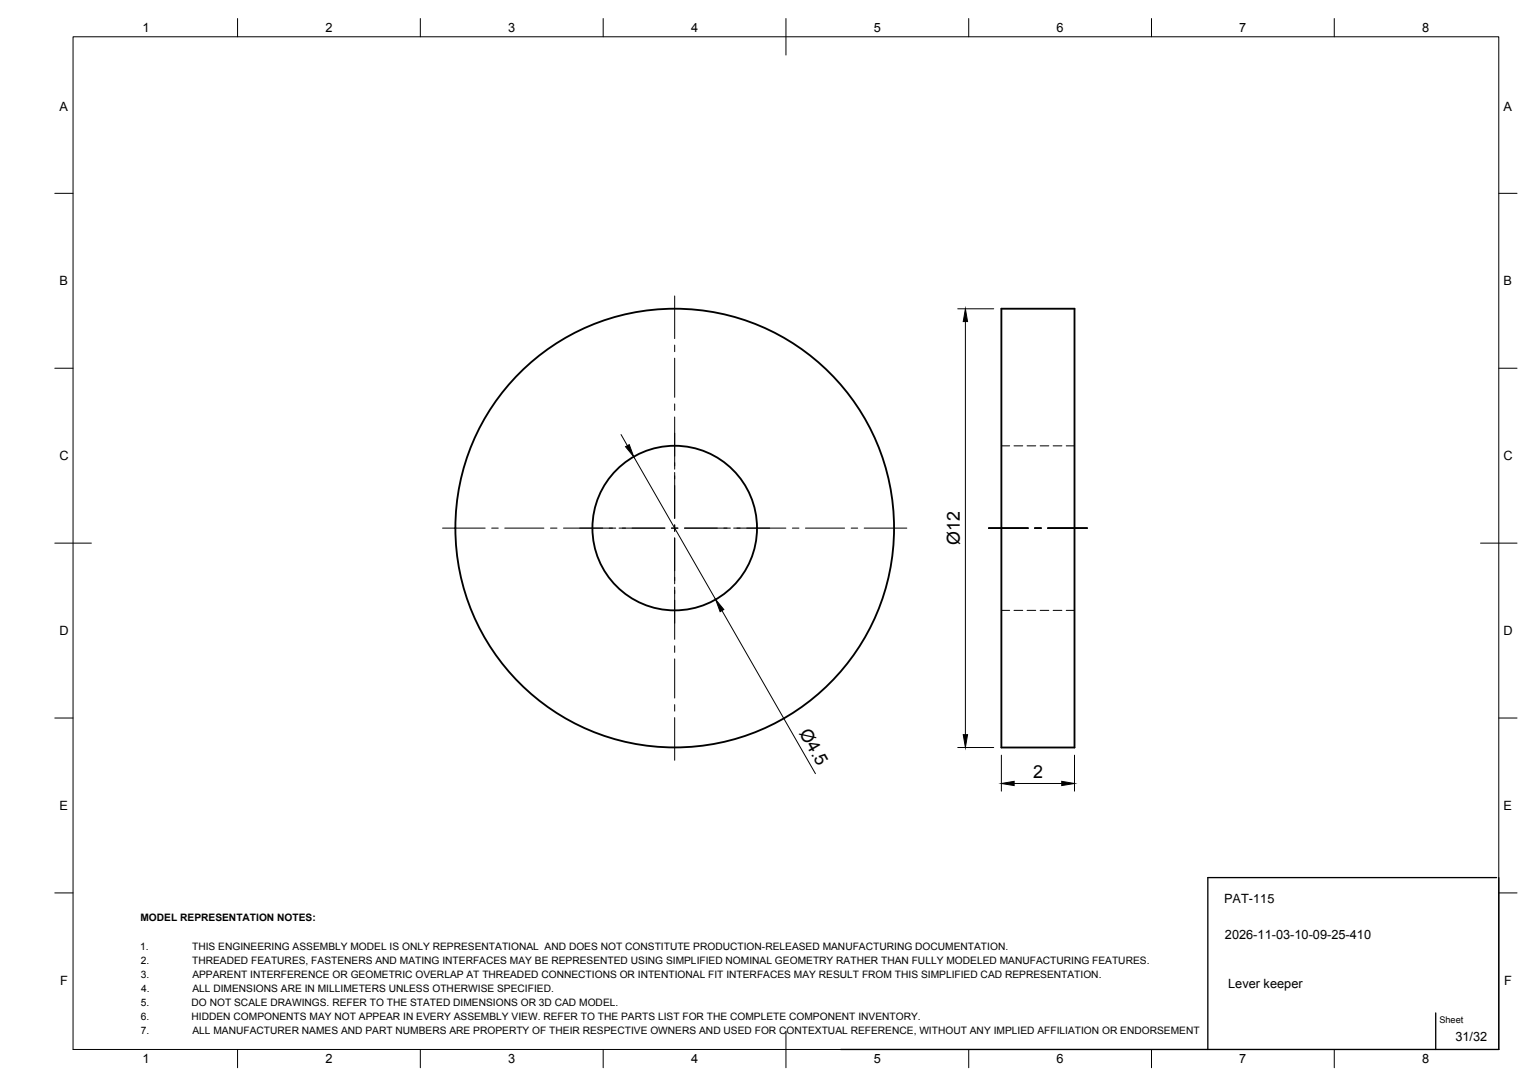
ISO-10303-21;
HEADER;
/* Generated by software containing ST-Developer
 * from STEP Tools, Inc. (www.steptools.com) 
 */

FILE_DESCRIPTION(
/* description */ ('Union bypass pipe loop'),
/* implementation_level */ '2;1');

FILE_NAME(
/* name */ 'Lever keeper.step',
/* time_stamp */ '2026-10-27T21:00:29-07:00',
/* author */ (''),
/* organization */ (''),
/* preprocessor_version */ 'ST-DEVELOPER v20.2',
/* originating_system */ 'Autodesk Translation Framework v15.17.0.0',
/* authorisation */ '');

FILE_SCHEMA (('AUTOMOTIVE_DESIGN { 1 0 10303 214 3 1 1 }'));
ENDSEC;

DATA;
#10=MECHANICAL_DESIGN_GEOMETRIC_PRESENTATION_REPRESENTATION('',(#474),#10095);
#410=SHAPE_REPRESENTATION_RELATIONSHIP('SRR','None',#10280,#442);
#442=ADVANCED_BREP_SHAPE_REPRESENTATION('',(#503),#10092);
#474=STYLED_ITEM('',(#10493),#503);
#503=MANIFOLD_SOLID_BREP('Body1',#5548);
#632=FACE_BOUND('',#1597,.T.);
#633=FACE_BOUND('',#1599,.T.);
#816=PLANE('',#6578);
#817=PLANE('',#6579);
#1141=FACE_OUTER_BOUND('',#1594,.T.);
#1142=FACE_OUTER_BOUND('',#1595,.T.);
#1143=FACE_OUTER_BOUND('',#1596,.T.);
#1144=FACE_OUTER_BOUND('',#1598,.T.);
#1594=EDGE_LOOP('',(#4984,#4985,#4986,#4987));
#1595=EDGE_LOOP('',(#4988,#4989,#4990,#4991));
#1596=EDGE_LOOP('',(#4992));
#1597=EDGE_LOOP('',(#4993));
#1598=EDGE_LOOP('',(#4994));
#1599=EDGE_LOOP('',(#4995));
#1962=LINE('',#9911,#2338);
#1963=LINE('',#9917,#2339);
#2338=VECTOR('',#8296,0.225);
#2339=VECTOR('',#8303,0.6);
#2619=CIRCLE('',#6573,0.225);
#2620=CIRCLE('',#6574,0.225);
#2621=CIRCLE('',#6576,0.6);
#2622=CIRCLE('',#6577,0.6);
#3036=VERTEX_POINT('',#9908);
#3037=VERTEX_POINT('',#9910);
#3038=VERTEX_POINT('',#9914);
#3039=VERTEX_POINT('',#9916);
#3690=EDGE_CURVE('',#3036,#3036,#2619,.T.);
#3691=EDGE_CURVE('',#3036,#3037,#1962,.T.);
#3692=EDGE_CURVE('',#3037,#3037,#2620,.T.);
#3693=EDGE_CURVE('',#3038,#3038,#2621,.T.);
#3694=EDGE_CURVE('',#3038,#3039,#1963,.T.);
#3695=EDGE_CURVE('',#3039,#3039,#2622,.T.);
#4984=ORIENTED_EDGE('',*,*,#3690,.F.);
#4985=ORIENTED_EDGE('',*,*,#3691,.T.);
#4986=ORIENTED_EDGE('',*,*,#3692,.T.);
#4987=ORIENTED_EDGE('',*,*,#3691,.F.);
#4988=ORIENTED_EDGE('',*,*,#3693,.F.);
#4989=ORIENTED_EDGE('',*,*,#3694,.T.);
#4990=ORIENTED_EDGE('',*,*,#3695,.T.);
#4991=ORIENTED_EDGE('',*,*,#3694,.F.);
#4992=ORIENTED_EDGE('',*,*,#3693,.T.);
#4993=ORIENTED_EDGE('',*,*,#3690,.T.);
#4994=ORIENTED_EDGE('',*,*,#3695,.F.);
#4995=ORIENTED_EDGE('',*,*,#3692,.F.);
#5180=CYLINDRICAL_SURFACE('',#6572,0.225);
#5181=CYLINDRICAL_SURFACE('',#6575,0.6);
#5490=ADVANCED_FACE('',(#1141),#5180,.F.);
#5491=ADVANCED_FACE('',(#1142),#5181,.T.);
#5492=ADVANCED_FACE('',(#1143,#632),#816,.T.);
#5493=ADVANCED_FACE('',(#1144,#633),#817,.F.);
#5548=CLOSED_SHELL('',(#5490,#5491,#5492,#5493));
#6571=AXIS2_PLACEMENT_3D('',#9906,#8290,#8291);
#6572=AXIS2_PLACEMENT_3D('',#9907,#8292,#8293);
#6573=AXIS2_PLACEMENT_3D('',#9909,#8294,#8295);
#6574=AXIS2_PLACEMENT_3D('',#9912,#8297,#8298);
#6575=AXIS2_PLACEMENT_3D('',#9913,#8299,#8300);
#6576=AXIS2_PLACEMENT_3D('',#9915,#8301,#8302);
#6577=AXIS2_PLACEMENT_3D('',#9918,#8304,#8305);
#6578=AXIS2_PLACEMENT_3D('',#9919,#8306,#8307);
#6579=AXIS2_PLACEMENT_3D('',#9920,#8308,#8309);
#8290=DIRECTION('axis',(0.,0.,1.));
#8291=DIRECTION('refdir',(1.,0.,0.));
#8292=DIRECTION('center_axis',(0.,0.,1.));
#8293=DIRECTION('ref_axis',(1.,0.,0.));
#8294=DIRECTION('center_axis',(0.,0.,-1.));
#8295=DIRECTION('ref_axis',(1.,0.,0.));
#8296=DIRECTION('',(0.,0.,-1.));
#8297=DIRECTION('center_axis',(0.,0.,-1.));
#8298=DIRECTION('ref_axis',(1.,0.,0.));
#8299=DIRECTION('center_axis',(0.,0.,1.));
#8300=DIRECTION('ref_axis',(1.,0.,0.));
#8301=DIRECTION('center_axis',(0.,0.,1.));
#8302=DIRECTION('ref_axis',(1.,0.,0.));
#8303=DIRECTION('',(0.,0.,-1.));
#8304=DIRECTION('center_axis',(0.,0.,1.));
#8305=DIRECTION('ref_axis',(1.,0.,0.));
#8306=DIRECTION('center_axis',(0.,0.,1.));
#8307=DIRECTION('ref_axis',(1.,0.,0.));
#8308=DIRECTION('center_axis',(0.,0.,1.));
#8309=DIRECTION('ref_axis',(1.,0.,0.));
#9906=CARTESIAN_POINT('',(0.,0.,0.));
#9907=CARTESIAN_POINT('Origin',(0.,0.,9.4));
#9908=CARTESIAN_POINT('',(-0.225,-2.75545529808154E-17,9.6));
#9909=CARTESIAN_POINT('Origin',(0.,0.,9.6));
#9910=CARTESIAN_POINT('',(-0.225,-2.75545529808154E-17,9.4));
#9911=CARTESIAN_POINT('',(-0.225,-2.75545529808154E-17,9.4));
#9912=CARTESIAN_POINT('Origin',(0.,0.,9.4));
#9913=CARTESIAN_POINT('Origin',(0.,0.,9.4));
#9914=CARTESIAN_POINT('',(-0.6,-7.34788079488412E-17,9.6));
#9915=CARTESIAN_POINT('Origin',(0.,0.,9.6));
#9916=CARTESIAN_POINT('',(-0.6,-7.34788079488412E-17,9.4));
#9917=CARTESIAN_POINT('',(-0.6,-7.34788079488412E-17,9.4));
#9918=CARTESIAN_POINT('Origin',(0.,0.,9.4));
#9919=CARTESIAN_POINT('Origin',(0.,0.,9.6));
#9920=CARTESIAN_POINT('Origin',(0.,0.,9.4));
#10055=UNCERTAINTY_MEASURE_WITH_UNIT(LENGTH_MEASURE(0.001),#10096,
'DISTANCE_ACCURACY_VALUE',
'Maximum model space distance between geometric entities at asserted c
onnectivities');
#10058=UNCERTAINTY_MEASURE_WITH_UNIT(LENGTH_MEASURE(0.001),#10096,
'DISTANCE_ACCURACY_VALUE',
'Maximum model space distance between geometric entities at asserted c
onnectivities');
#10092=(
GEOMETRIC_REPRESENTATION_CONTEXT(3)
GLOBAL_UNCERTAINTY_ASSIGNED_CONTEXT((#10055))
GLOBAL_UNIT_ASSIGNED_CONTEXT((#10096,#10098,#10099))
REPRESENTATION_CONTEXT('','3D')
);
#10095=(
GEOMETRIC_REPRESENTATION_CONTEXT(3)
GLOBAL_UNCERTAINTY_ASSIGNED_CONTEXT((#10058))
GLOBAL_UNIT_ASSIGNED_CONTEXT((#10096,#10098,#10099))
REPRESENTATION_CONTEXT('','3D')
);
#10096=(
LENGTH_UNIT()
NAMED_UNIT(*)
SI_UNIT(.CENTI.,.METRE.)
);
#10098=(
NAMED_UNIT(*)
PLANE_ANGLE_UNIT()
SI_UNIT($,.RADIAN.)
);
#10099=(
NAMED_UNIT(*)
SI_UNIT($,.STERADIAN.)
SOLID_ANGLE_UNIT()
);
#10133=SHAPE_DEFINITION_REPRESENTATION(#10236,#10280);
#10236=PRODUCT_DEFINITION_SHAPE('',$,#10317);
#10280=SHAPE_REPRESENTATION('',(#6571),#10092);
#10283=PRODUCT_DEFINITION_CONTEXT('part definition',#10393,'design');
#10317=PRODUCT_DEFINITION('Lever keeper','Lever keeper',#10353,#10283);
#10353=PRODUCT_DEFINITION_FORMATION('',$,#10428);
#10393=APPLICATION_CONTEXT(
'Core Data for Automotive Mechanical Design Process');
#10394=PRODUCT_CONTEXT('part definition',#10393,'mechanical');
#10428=PRODUCT('Lever keeper','Lever keeper','Lever keeper',(#10394));
#10487=COLOUR_RGB('Sky Blue',0.24,0.69,0.87);
#10488=FILL_AREA_STYLE_COLOUR('',#10487);
#10489=FILL_AREA_STYLE('',(#10488));
#10490=SURFACE_STYLE_FILL_AREA(#10489);
#10491=SURFACE_SIDE_STYLE('',(#10490));
#10492=SURFACE_STYLE_USAGE(.BOTH.,#10491);
#10493=PRESENTATION_STYLE_ASSIGNMENT((#10492));
ENDSEC;
END-ISO-10303-21;
